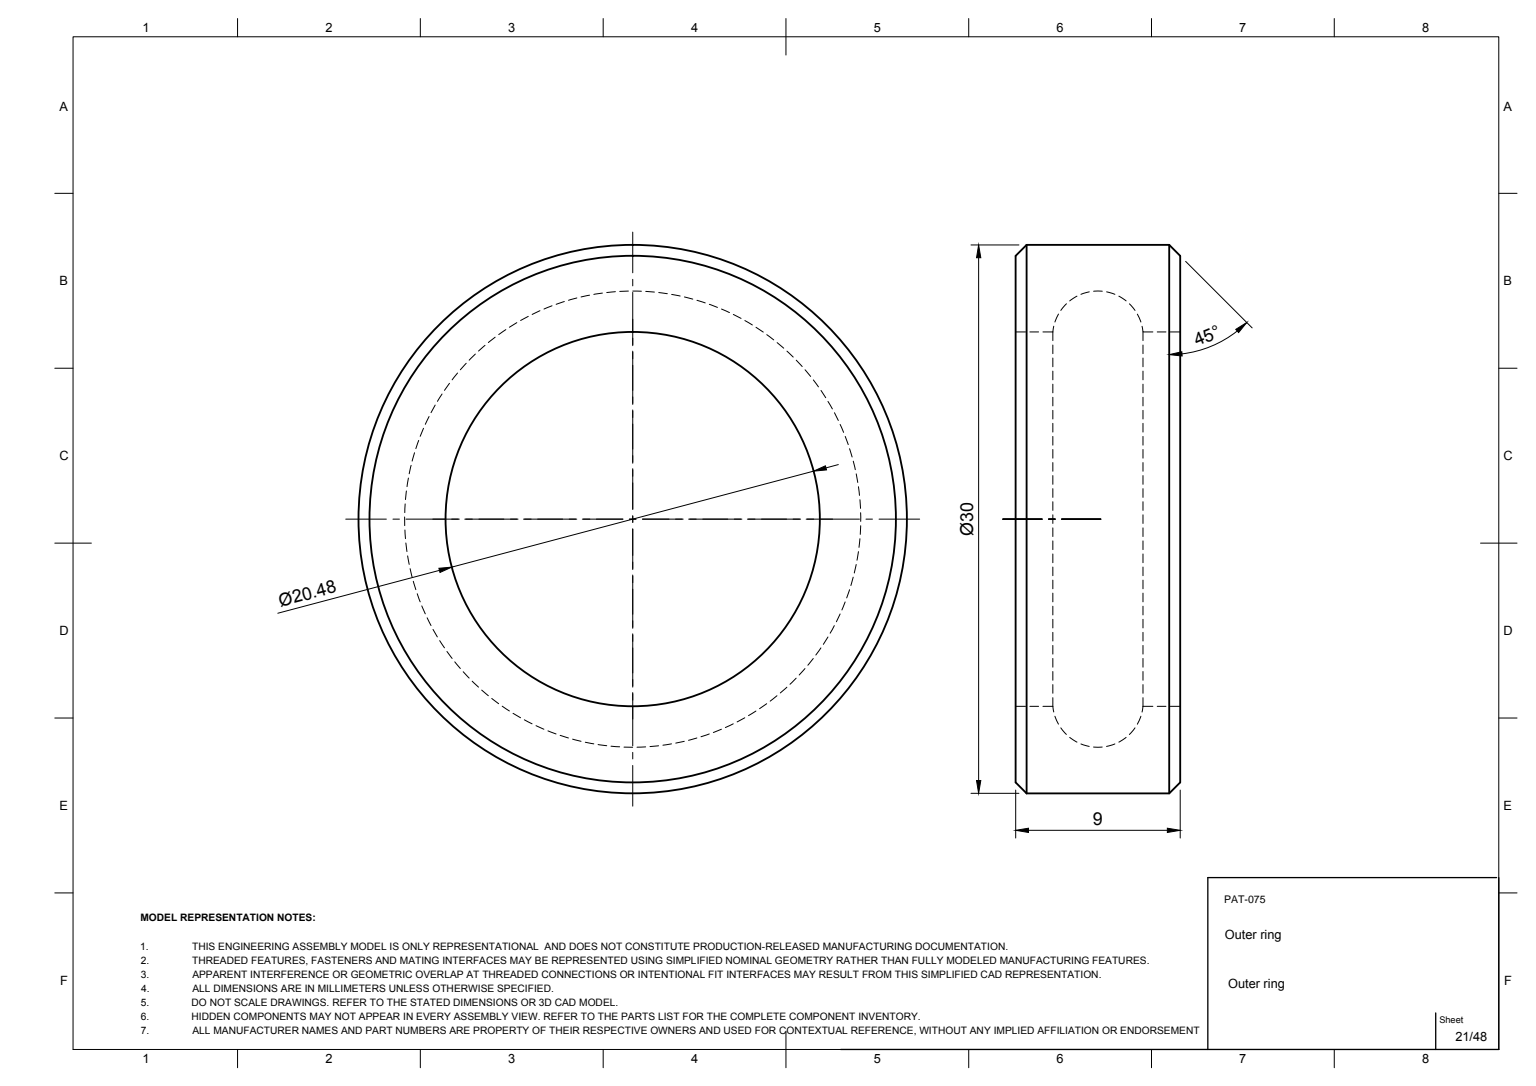
ISO-10303-21;
HEADER;
/* Generated by software containing ST-Developer
 * from STEP Tools, Inc. (www.steptools.com) 
 */

FILE_DESCRIPTION(
/* description */ ('Over-Centre Plunger Toggle Clamp on Slotted Fixture Frame'),
/* implementation_level */ '2;1');

FILE_NAME(
/* name */ 
'Outer ring.step',
/* time_stamp */ '2026-10-28T03:23:24-07:00',
/* author */ (''),
/* organization */ (''),
/* preprocessor_version */ 'ST-DEVELOPER v20.2',
/* originating_system */ 'Autodesk Translation Framework v15.17.0.0',
/* authorisation */ '');

FILE_SCHEMA (('AUTOMOTIVE_DESIGN { 1 0 10303 214 3 1 1 }'));
ENDSEC;

DATA;
#10=MECHANICAL_DESIGN_GEOMETRIC_PRESENTATION_REPRESENTATION('',(#530),#15212);
#396=TOROIDAL_SURFACE('',#9186,1.,0.247676);
#411=CONICAL_SURFACE('',#9197,1.47,0.785398163397449);
#412=CONICAL_SURFACE('',#9201,1.47,0.785398163397449);
#446=SHAPE_REPRESENTATION_RELATIONSHIP('SRR','None',#15421,#488);
#488=ADVANCED_BREP_SHAPE_REPRESENTATION('',(#580),#15183);
#530=STYLED_ITEM('',(#15719),#580);
#580=MANIFOLD_SOLID_BREP('Body1',#8263);
#722=FACE_BOUND('',#1926,.T.);
#723=FACE_BOUND('',#1931,.T.);
#940=PLANE('',#9194);
#941=PLANE('',#9203);
#1326=FACE_OUTER_BOUND('',#1923,.T.);
#1327=FACE_OUTER_BOUND('',#1924,.T.);
#1328=FACE_OUTER_BOUND('',#1925,.T.);
#1329=FACE_OUTER_BOUND('',#1927,.T.);
#1330=FACE_OUTER_BOUND('',#1928,.T.);
#1331=FACE_OUTER_BOUND('',#1929,.T.);
#1332=FACE_OUTER_BOUND('',#1930,.T.);
#1333=FACE_OUTER_BOUND('',#1932,.T.);
#1923=EDGE_LOOP('',(#6661,#6662,#6663,#6664,#6665,#6666));
#1924=EDGE_LOOP('',(#6667,#6668,#6669,#6670,#6671));
#1925=EDGE_LOOP('',(#6672));
#1926=EDGE_LOOP('',(#6673));
#1927=EDGE_LOOP('',(#6674,#6675,#6676,#6677));
#1928=EDGE_LOOP('',(#6678,#6679,#6680,#6681));
#1929=EDGE_LOOP('',(#6682,#6683,#6684,#6685));
#1930=EDGE_LOOP('',(#6686));
#1931=EDGE_LOOP('',(#6687));
#1932=EDGE_LOOP('',(#6688,#6689,#6690,#6691,#6692));
#2614=LINE('',#13547,#3244);
#2615=LINE('',#13556,#3245);
#2616=LINE('',#13560,#3246);
#2617=LINE('',#13564,#3247);
#2618=LINE('',#13567,#3248);
#3244=VECTOR('',#10999,1.023815);
#3245=VECTOR('',#11010,1.47);
#3246=VECTOR('',#11015,1.5);
#3247=VECTOR('',#11020,1.47);
#3248=VECTOR('',#11025,1.023815);
#3652=CIRCLE('',#9187,1.023815);
#3653=CIRCLE('',#9188,1.023815);
#3654=CIRCLE('',#9189,0.247676);
#3655=CIRCLE('',#9190,1.023815);
#3656=CIRCLE('',#9191,1.023815);
#3657=CIRCLE('',#9193,1.023815);
#3658=CIRCLE('',#9195,1.44);
#3659=CIRCLE('',#9196,1.023815);
#3660=CIRCLE('',#9198,1.5);
#3661=CIRCLE('',#9200,1.5);
#3662=CIRCLE('',#9202,1.44);
#4221=VERTEX_POINT('',#13535);
#4222=VERTEX_POINT('',#13536);
#4223=VERTEX_POINT('',#13539);
#4224=VERTEX_POINT('',#13541);
#4225=VERTEX_POINT('',#13545);
#4226=VERTEX_POINT('',#13549);
#4227=VERTEX_POINT('',#13551);
#4228=VERTEX_POINT('',#13554);
#4229=VERTEX_POINT('',#13558);
#4230=VERTEX_POINT('',#13562);
#5091=EDGE_CURVE('',#4221,#4222,#3652,.T.);
#5092=EDGE_CURVE('',#4222,#4221,#3653,.T.);
#5093=EDGE_CURVE('',#4222,#4223,#3654,.T.);
#5094=EDGE_CURVE('',#4224,#4223,#3655,.T.);
#5095=EDGE_CURVE('',#4223,#4224,#3656,.T.);
#5096=EDGE_CURVE('',#4225,#4225,#3657,.T.);
#5097=EDGE_CURVE('',#4225,#4224,#2614,.T.);
#5098=EDGE_CURVE('',#4226,#4226,#3658,.T.);
#5099=EDGE_CURVE('',#4227,#4227,#3659,.T.);
#5100=EDGE_CURVE('',#4228,#4228,#3660,.T.);
#5101=EDGE_CURVE('',#4228,#4226,#2615,.T.);
#5102=EDGE_CURVE('',#4229,#4229,#3661,.T.);
#5103=EDGE_CURVE('',#4229,#4228,#2616,.T.);
#5104=EDGE_CURVE('',#4230,#4230,#3662,.T.);
#5105=EDGE_CURVE('',#4230,#4229,#2617,.T.);
#5106=EDGE_CURVE('',#4221,#4227,#2618,.T.);
#6661=ORIENTED_EDGE('',*,*,#5091,.F.);
#6662=ORIENTED_EDGE('',*,*,#5092,.F.);
#6663=ORIENTED_EDGE('',*,*,#5093,.T.);
#6664=ORIENTED_EDGE('',*,*,#5094,.F.);
#6665=ORIENTED_EDGE('',*,*,#5095,.F.);
#6666=ORIENTED_EDGE('',*,*,#5093,.F.);
#6667=ORIENTED_EDGE('',*,*,#5096,.T.);
#6668=ORIENTED_EDGE('',*,*,#5097,.T.);
#6669=ORIENTED_EDGE('',*,*,#5094,.T.);
#6670=ORIENTED_EDGE('',*,*,#5095,.T.);
#6671=ORIENTED_EDGE('',*,*,#5097,.F.);
#6672=ORIENTED_EDGE('',*,*,#5098,.F.);
#6673=ORIENTED_EDGE('',*,*,#5099,.T.);
#6674=ORIENTED_EDGE('',*,*,#5100,.F.);
#6675=ORIENTED_EDGE('',*,*,#5101,.T.);
#6676=ORIENTED_EDGE('',*,*,#5098,.T.);
#6677=ORIENTED_EDGE('',*,*,#5101,.F.);
#6678=ORIENTED_EDGE('',*,*,#5102,.F.);
#6679=ORIENTED_EDGE('',*,*,#5103,.T.);
#6680=ORIENTED_EDGE('',*,*,#5100,.T.);
#6681=ORIENTED_EDGE('',*,*,#5103,.F.);
#6682=ORIENTED_EDGE('',*,*,#5104,.F.);
#6683=ORIENTED_EDGE('',*,*,#5105,.T.);
#6684=ORIENTED_EDGE('',*,*,#5102,.T.);
#6685=ORIENTED_EDGE('',*,*,#5105,.F.);
#6686=ORIENTED_EDGE('',*,*,#5104,.T.);
#6687=ORIENTED_EDGE('',*,*,#5096,.F.);
#6688=ORIENTED_EDGE('',*,*,#5091,.T.);
#6689=ORIENTED_EDGE('',*,*,#5092,.T.);
#6690=ORIENTED_EDGE('',*,*,#5106,.T.);
#6691=ORIENTED_EDGE('',*,*,#5099,.F.);
#6692=ORIENTED_EDGE('',*,*,#5106,.F.);
#7692=CYLINDRICAL_SURFACE('',#9192,1.023815);
#7693=CYLINDRICAL_SURFACE('',#9199,1.5);
#7694=CYLINDRICAL_SURFACE('',#9204,1.023815);
#7998=ADVANCED_FACE('',(#1326),#396,.F.);
#7999=ADVANCED_FACE('',(#1327),#7692,.F.);
#8000=ADVANCED_FACE('',(#1328,#722),#940,.T.);
#8001=ADVANCED_FACE('',(#1329),#411,.T.);
#8002=ADVANCED_FACE('',(#1330),#7693,.T.);
#8003=ADVANCED_FACE('',(#1331),#412,.T.);
#8004=ADVANCED_FACE('',(#1332,#723),#941,.T.);
#8005=ADVANCED_FACE('',(#1333),#7694,.F.);
#8263=CLOSED_SHELL('',(#7998,#7999,#8000,#8001,#8002,#8003,#8004,#8005));
#9185=AXIS2_PLACEMENT_3D('',#13533,#10981,#10982);
#9186=AXIS2_PLACEMENT_3D('',#13534,#10983,#10984);
#9187=AXIS2_PLACEMENT_3D('',#13537,#10985,#10986);
#9188=AXIS2_PLACEMENT_3D('',#13538,#10987,#10988);
#9189=AXIS2_PLACEMENT_3D('',#13540,#10989,#10990);
#9190=AXIS2_PLACEMENT_3D('',#13542,#10991,#10992);
#9191=AXIS2_PLACEMENT_3D('',#13543,#10993,#10994);
#9192=AXIS2_PLACEMENT_3D('',#13544,#10995,#10996);
#9193=AXIS2_PLACEMENT_3D('',#13546,#10997,#10998);
#9194=AXIS2_PLACEMENT_3D('',#13548,#11000,#11001);
#9195=AXIS2_PLACEMENT_3D('',#13550,#11002,#11003);
#9196=AXIS2_PLACEMENT_3D('',#13552,#11004,#11005);
#9197=AXIS2_PLACEMENT_3D('',#13553,#11006,#11007);
#9198=AXIS2_PLACEMENT_3D('',#13555,#11008,#11009);
#9199=AXIS2_PLACEMENT_3D('',#13557,#11011,#11012);
#9200=AXIS2_PLACEMENT_3D('',#13559,#11013,#11014);
#9201=AXIS2_PLACEMENT_3D('',#13561,#11016,#11017);
#9202=AXIS2_PLACEMENT_3D('',#13563,#11018,#11019);
#9203=AXIS2_PLACEMENT_3D('',#13565,#11021,#11022);
#9204=AXIS2_PLACEMENT_3D('',#13566,#11023,#11024);
#10981=DIRECTION('axis',(0.,0.,1.));
#10982=DIRECTION('refdir',(1.,0.,0.));
#10983=DIRECTION('center_axis',(0.,-1.,0.));
#10984=DIRECTION('ref_axis',(0.,0.,-1.));
#10985=DIRECTION('center_axis',(0.,-1.,0.));
#10986=DIRECTION('ref_axis',(1.,0.,0.));
#10987=DIRECTION('center_axis',(0.,-1.,0.));
#10988=DIRECTION('ref_axis',(1.,0.,0.));
#10989=DIRECTION('center_axis',(1.,0.,1.22464679914735E-16));
#10990=DIRECTION('ref_axis',(-1.22464679914735E-16,0.,1.));
#10991=DIRECTION('center_axis',(0.,1.,0.));
#10992=DIRECTION('ref_axis',(1.,0.,0.));
#10993=DIRECTION('center_axis',(0.,1.,0.));
#10994=DIRECTION('ref_axis',(1.,0.,0.));
#10995=DIRECTION('center_axis',(0.,-1.,0.));
#10996=DIRECTION('ref_axis',(1.,0.,0.));
#10997=DIRECTION('center_axis',(0.,-1.,0.));
#10998=DIRECTION('ref_axis',(1.,0.,0.));
#10999=DIRECTION('',(0.,1.,0.));
#11000=DIRECTION('center_axis',(0.,1.,0.));
#11001=DIRECTION('ref_axis',(0.,0.,1.));
#11002=DIRECTION('center_axis',(0.,-1.,0.));
#11003=DIRECTION('ref_axis',(1.,0.,0.));
#11004=DIRECTION('center_axis',(0.,-1.,0.));
#11005=DIRECTION('ref_axis',(1.,0.,0.));
#11006=DIRECTION('center_axis',(0.,-1.,0.));
#11007=DIRECTION('ref_axis',(1.,0.,0.));
#11008=DIRECTION('center_axis',(0.,-1.,0.));
#11009=DIRECTION('ref_axis',(1.,0.,0.));
#11010=DIRECTION('',(0.707106781186548,0.707106781186547,8.65956056235494E-17));
#11011=DIRECTION('center_axis',(0.,-1.,0.));
#11012=DIRECTION('ref_axis',(1.,0.,0.));
#11013=DIRECTION('center_axis',(0.,-1.,0.));
#11014=DIRECTION('ref_axis',(1.,0.,0.));
#11015=DIRECTION('',(0.,1.,0.));
#11016=DIRECTION('center_axis',(0.,1.,0.));
#11017=DIRECTION('ref_axis',(1.,0.,0.));
#11018=DIRECTION('center_axis',(0.,-1.,0.));
#11019=DIRECTION('ref_axis',(1.,0.,0.));
#11020=DIRECTION('',(-0.707106781186548,0.707106781186547,-8.65956056235494E-17));
#11021=DIRECTION('center_axis',(0.,-1.,0.));
#11022=DIRECTION('ref_axis',(0.,0.,-1.));
#11023=DIRECTION('center_axis',(0.,-1.,0.));
#11024=DIRECTION('ref_axis',(1.,0.,0.));
#11025=DIRECTION('',(0.,1.,0.));
#13533=CARTESIAN_POINT('',(0.,0.,0.));
#13534=CARTESIAN_POINT('Origin',(0.,0.,0.));
#13535=CARTESIAN_POINT('',(-1.023815,0.246528389340863,-1.25381176266905E-16));
#13536=CARTESIAN_POINT('',(-1.25381176266905E-16,0.246528389340863,1.023815));
#13537=CARTESIAN_POINT('Origin',(0.,0.246528389340863,0.));
#13538=CARTESIAN_POINT('Origin',(0.,0.246528389340863,0.));
#13539=CARTESIAN_POINT('',(-1.25381176266905E-16,-0.246528389340863,1.023815));
#13540=CARTESIAN_POINT('Origin',(-1.22464679914735E-16,0.,1.));
#13541=CARTESIAN_POINT('',(-1.023815,-0.246528389340863,1.25381176266905E-16));
#13542=CARTESIAN_POINT('Origin',(0.,-0.246528389340863,0.));
#13543=CARTESIAN_POINT('Origin',(0.,-0.246528389340863,0.));
#13544=CARTESIAN_POINT('Origin',(0.,0.,0.));
#13545=CARTESIAN_POINT('',(-1.023815,-0.45,-1.25381176266905E-16));
#13546=CARTESIAN_POINT('Origin',(0.,-0.45,0.));
#13547=CARTESIAN_POINT('',(-1.023815,0.,-1.25381176266905E-16));
#13548=CARTESIAN_POINT('Origin',(1.44,0.45,0.));
#13549=CARTESIAN_POINT('',(-1.44,0.45,-1.76349139077219E-16));
#13550=CARTESIAN_POINT('Origin',(0.,0.45,0.));
#13551=CARTESIAN_POINT('',(-1.023815,0.45,-1.25381176266905E-16));
#13552=CARTESIAN_POINT('Origin',(0.,0.45,0.));
#13553=CARTESIAN_POINT('Origin',(0.,0.42,0.));
#13554=CARTESIAN_POINT('',(-1.5,0.39,-1.83697019872103E-16));
#13555=CARTESIAN_POINT('Origin',(0.,0.39,0.));
#13556=CARTESIAN_POINT('',(-1.47,0.42,-1.80023079474661E-16));
#13557=CARTESIAN_POINT('Origin',(0.,0.,0.));
#13558=CARTESIAN_POINT('',(-1.5,-0.39,-1.83697019872103E-16));
#13559=CARTESIAN_POINT('Origin',(0.,-0.39,0.));
#13560=CARTESIAN_POINT('',(-1.5,0.,-1.83697019872103E-16));
#13561=CARTESIAN_POINT('Origin',(0.,-0.42,0.));
#13562=CARTESIAN_POINT('',(-1.44,-0.45,-1.76349139077219E-16));
#13563=CARTESIAN_POINT('Origin',(0.,-0.45,0.));
#13564=CARTESIAN_POINT('',(-1.47,-0.42,-1.80023079474661E-16));
#13565=CARTESIAN_POINT('Origin',(1.023815,-0.45,0.));
#13566=CARTESIAN_POINT('Origin',(0.,0.,0.));
#13567=CARTESIAN_POINT('',(-1.023815,0.,-1.25381176266905E-16));
#15133=UNCERTAINTY_MEASURE_WITH_UNIT(LENGTH_MEASURE(0.001),#15213,
'DISTANCE_ACCURACY_VALUE',
'Maximum model space distance between geometric entities at asserted c
onnectivities');
#15162=UNCERTAINTY_MEASURE_WITH_UNIT(LENGTH_MEASURE(0.001),#15213,
'DISTANCE_ACCURACY_VALUE',
'Maximum model space distance between geometric entities at asserted c
onnectivities');
#15183=(
GEOMETRIC_REPRESENTATION_CONTEXT(3)
GLOBAL_UNCERTAINTY_ASSIGNED_CONTEXT((#15133))
GLOBAL_UNIT_ASSIGNED_CONTEXT((#15213,#15215,#15216))
REPRESENTATION_CONTEXT('','3D')
);
#15212=(
GEOMETRIC_REPRESENTATION_CONTEXT(3)
GLOBAL_UNCERTAINTY_ASSIGNED_CONTEXT((#15162))
GLOBAL_UNIT_ASSIGNED_CONTEXT((#15213,#15215,#15216))
REPRESENTATION_CONTEXT('','3D')
);
#15213=(
LENGTH_UNIT()
NAMED_UNIT(*)
SI_UNIT(.CENTI.,.METRE.)
);
#15215=(
NAMED_UNIT(*)
PLANE_ANGLE_UNIT()
SI_UNIT($,.RADIAN.)
);
#15216=(
NAMED_UNIT(*)
SI_UNIT($,.STERADIAN.)
SOLID_ANGLE_UNIT()
);
#15237=SHAPE_DEFINITION_REPRESENTATION(#15286,#15421);
#15286=PRODUCT_DEFINITION_SHAPE('',$,#15471);
#15421=SHAPE_REPRESENTATION('',(#9185),#15183);
#15450=PRODUCT_DEFINITION_CONTEXT('part definition',#15599,'design');
#15471=PRODUCT_DEFINITION('Outer ring','Outer ring',#15520,#15450);
#15520=PRODUCT_DEFINITION_FORMATION('',$,#15621);
#15599=APPLICATION_CONTEXT(
'Core Data for Automotive Mechanical Design Process');
#15600=PRODUCT_CONTEXT('part definition',#15599,'mechanical');
#15621=PRODUCT('Outer ring','Outer ring','Outer ring',(#15600));
#15713=COLOUR_RGB('Grey',0.48,0.52,0.57);
#15714=FILL_AREA_STYLE_COLOUR('',#15713);
#15715=FILL_AREA_STYLE('',(#15714));
#15716=SURFACE_STYLE_FILL_AREA(#15715);
#15717=SURFACE_SIDE_STYLE('',(#15716));
#15718=SURFACE_STYLE_USAGE(.BOTH.,#15717);
#15719=PRESENTATION_STYLE_ASSIGNMENT((#15718));
ENDSEC;
END-ISO-10303-21;
